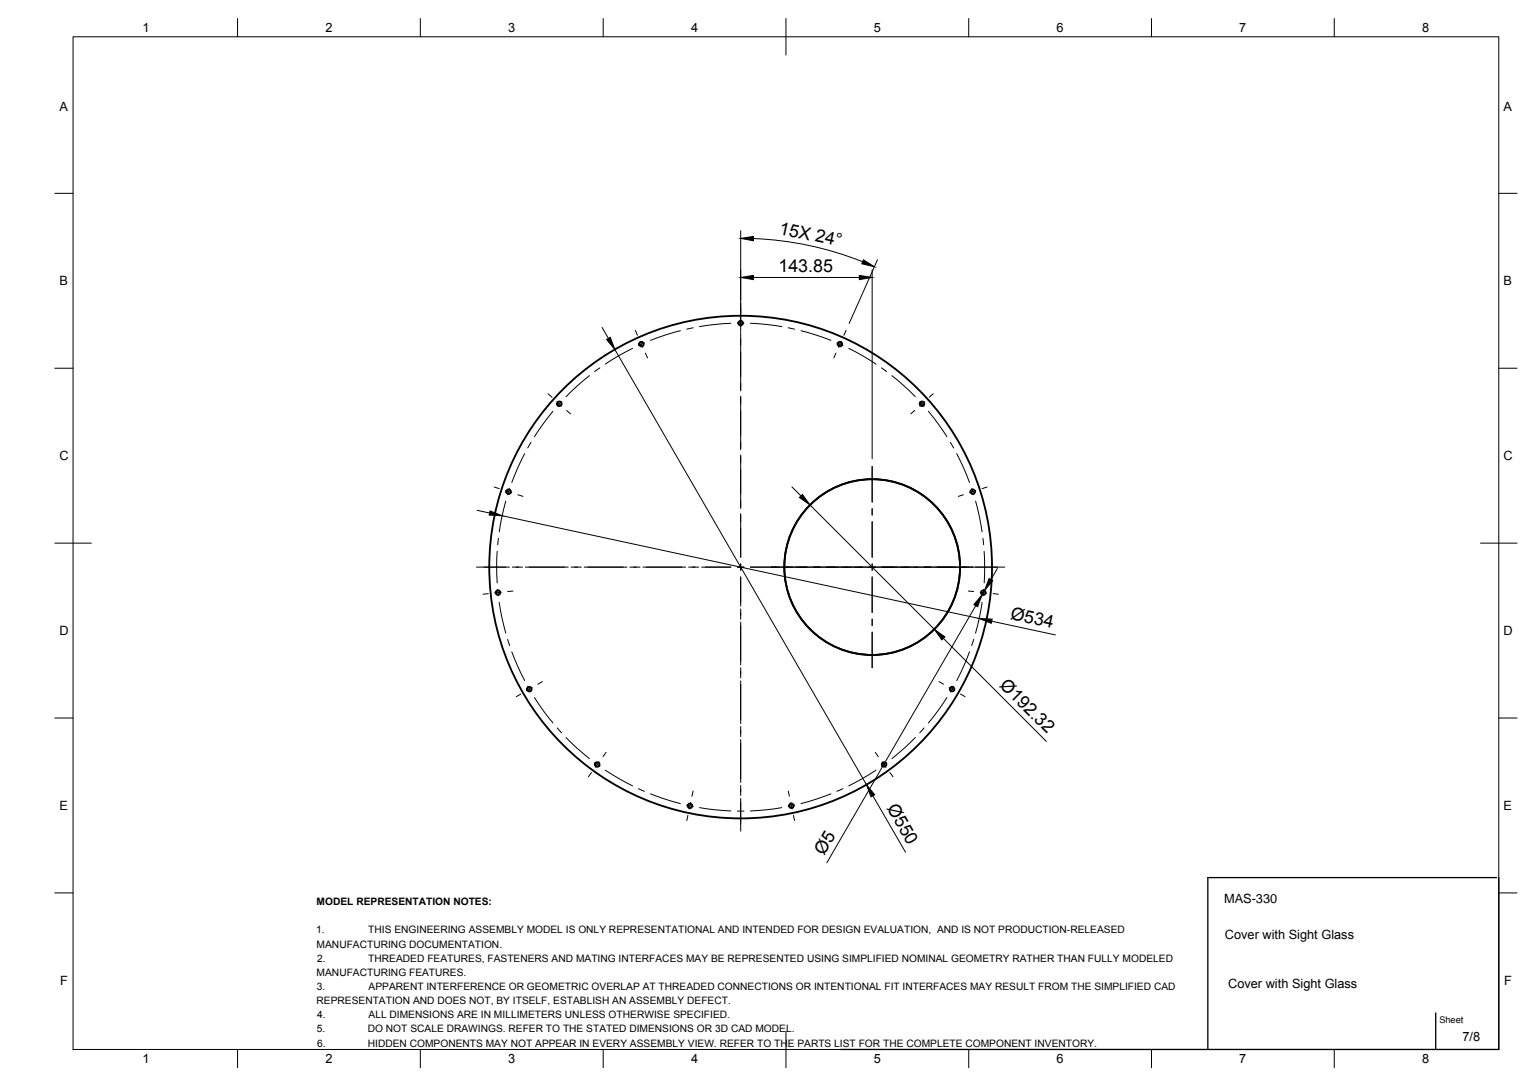
ISO-10303-21;
HEADER;
/* Generated by software containing ST-Developer
 * from STEP Tools, Inc. (www.steptools.com) 
 */

FILE_DESCRIPTION(
/* description */ ('STEP AP214'),
/* implementation_level */ '2;1');

FILE_NAME(
/* name */ 'Cover with Sight Glass.step',
/* time_stamp */ '2026-10-12T14:05:15-07:00',
/* author */ (''),
/* organization */ (''),
/* preprocessor_version */ 'ST-DEVELOPER v20.2',
/* originating_system */ 'Autodesk Translation Framework v15.15.0.0',
/* authorisation */ '');

FILE_SCHEMA (('AUTOMOTIVE_DESIGN { 1 0 10303 214 3 1 1 }'));
ENDSEC;

DATA;
#10=MECHANICAL_DESIGN_GEOMETRIC_PRESENTATION_REPRESENTATION('',(#286,#287),#39959);
#272=SHAPE_REPRESENTATION_RELATIONSHIP('SRR','None',#40006,#279);
#279=ADVANCED_BREP_SHAPE_REPRESENTATION('',(#294,#295),#39956);
#286=STYLED_ITEM('',(#40046),#294);
#287=STYLED_ITEM('',(#40046),#295);
#294=MANIFOLD_SOLID_BREP('Body1',#18263);
#295=MANIFOLD_SOLID_BREP('Body2',#18264);
#419=PLANE('',#18845);
#420=PLANE('',#18846);
#421=PLANE('',#18850);
#422=PLANE('',#18851);
#964=FACE_BOUND('',#6153,.T.);
#965=FACE_BOUND('',#6154,.T.);
#966=FACE_BOUND('',#6155,.T.);
#967=FACE_BOUND('',#6156,.T.);
#968=FACE_BOUND('',#6157,.T.);
#969=FACE_BOUND('',#6158,.T.);
#970=FACE_BOUND('',#6159,.T.);
#971=FACE_BOUND('',#6160,.T.);
#972=FACE_BOUND('',#6161,.T.);
#973=FACE_BOUND('',#6162,.T.);
#974=FACE_BOUND('',#6163,.T.);
#975=FACE_BOUND('',#6164,.T.);
#976=FACE_BOUND('',#6165,.T.);
#977=FACE_BOUND('',#6166,.T.);
#978=FACE_BOUND('',#6167,.T.);
#979=FACE_BOUND('',#6168,.T.);
#980=FACE_BOUND('',#6170,.T.);
#981=FACE_BOUND('',#6171,.T.);
#982=FACE_BOUND('',#6172,.T.);
#983=FACE_BOUND('',#6173,.T.);
#984=FACE_BOUND('',#6174,.T.);
#985=FACE_BOUND('',#6175,.T.);
#986=FACE_BOUND('',#6176,.T.);
#987=FACE_BOUND('',#6177,.T.);
#988=FACE_BOUND('',#6178,.T.);
#989=FACE_BOUND('',#6179,.T.);
#990=FACE_BOUND('',#6180,.T.);
#991=FACE_BOUND('',#6181,.T.);
#992=FACE_BOUND('',#6182,.T.);
#993=FACE_BOUND('',#6183,.T.);
#994=FACE_BOUND('',#6184,.T.);
#995=FACE_BOUND('',#6185,.T.);
#1772=LINE('',#30494,#3345);
#1773=LINE('',#30500,#3346);
#1774=LINE('',#30506,#3347);
#1775=LINE('',#30512,#3348);
#1776=LINE('',#30518,#3349);
#1777=LINE('',#30524,#3350);
#1778=LINE('',#30530,#3351);
#1779=LINE('',#30536,#3352);
#1780=LINE('',#30542,#3353);
#1781=LINE('',#30548,#3354);
#1782=LINE('',#30554,#3355);
#1783=LINE('',#30560,#3356);
#1784=LINE('',#30566,#3357);
#1785=LINE('',#30572,#3358);
#1786=LINE('',#30578,#3359);
#1787=LINE('',#30584,#3360);
#1788=LINE('',#30590,#3361);
#1789=LINE('',#30598,#3362);
#3345=VECTOR('',#21268,96.161193339026);
#3346=VECTOR('',#21275,2.5);
#3347=VECTOR('',#21282,2.5);
#3348=VECTOR('',#21289,2.5);
#3349=VECTOR('',#21296,2.5);
#3350=VECTOR('',#21303,2.5);
#3351=VECTOR('',#21310,2.5);
#3352=VECTOR('',#21317,2.5);
#3353=VECTOR('',#21324,2.5);
#3354=VECTOR('',#21331,2.50000000000001);
#3355=VECTOR('',#21338,2.5);
#3356=VECTOR('',#21345,2.5);
#3357=VECTOR('',#21352,2.5);
#3358=VECTOR('',#21359,2.5);
#3359=VECTOR('',#21366,2.5);
#3360=VECTOR('',#21373,2.5);
#3361=VECTOR('',#21380,275.);
#3362=VECTOR('',#21391,96.161193339026);
#4656=CYLINDRICAL_SURFACE('',#18794,96.161193339026);
#4657=CYLINDRICAL_SURFACE('',#18797,2.5);
#4658=CYLINDRICAL_SURFACE('',#18800,2.5);
#4659=CYLINDRICAL_SURFACE('',#18803,2.5);
#4660=CYLINDRICAL_SURFACE('',#18806,2.5);
#4661=CYLINDRICAL_SURFACE('',#18809,2.5);
#4662=CYLINDRICAL_SURFACE('',#18812,2.5);
#4663=CYLINDRICAL_SURFACE('',#18815,2.5);
#4664=CYLINDRICAL_SURFACE('',#18818,2.5);
#4665=CYLINDRICAL_SURFACE('',#18821,2.50000000000001);
#4666=CYLINDRICAL_SURFACE('',#18824,2.5);
#4667=CYLINDRICAL_SURFACE('',#18827,2.5);
#4668=CYLINDRICAL_SURFACE('',#18830,2.5);
#4669=CYLINDRICAL_SURFACE('',#18833,2.5);
#4670=CYLINDRICAL_SURFACE('',#18836,2.5);
#4671=CYLINDRICAL_SURFACE('',#18839,2.5);
#4672=CYLINDRICAL_SURFACE('',#18842,275.);
#4673=CYLINDRICAL_SURFACE('',#18847,96.161193339026);
#5054=FACE_OUTER_BOUND('',#6135,.T.);
#5055=FACE_OUTER_BOUND('',#6136,.T.);
#5056=FACE_OUTER_BOUND('',#6137,.T.);
#5057=FACE_OUTER_BOUND('',#6138,.T.);
#5058=FACE_OUTER_BOUND('',#6139,.T.);
#5059=FACE_OUTER_BOUND('',#6140,.T.);
#5060=FACE_OUTER_BOUND('',#6141,.T.);
#5061=FACE_OUTER_BOUND('',#6142,.T.);
#5062=FACE_OUTER_BOUND('',#6143,.T.);
#5063=FACE_OUTER_BOUND('',#6144,.T.);
#5064=FACE_OUTER_BOUND('',#6145,.T.);
#5065=FACE_OUTER_BOUND('',#6146,.T.);
#5066=FACE_OUTER_BOUND('',#6147,.T.);
#5067=FACE_OUTER_BOUND('',#6148,.T.);
#5068=FACE_OUTER_BOUND('',#6149,.T.);
#5069=FACE_OUTER_BOUND('',#6150,.T.);
#5070=FACE_OUTER_BOUND('',#6151,.T.);
#5071=FACE_OUTER_BOUND('',#6152,.T.);
#5072=FACE_OUTER_BOUND('',#6169,.T.);
#5073=FACE_OUTER_BOUND('',#6186,.T.);
#5074=FACE_OUTER_BOUND('',#6187,.T.);
#5075=FACE_OUTER_BOUND('',#6188,.T.);
#6135=EDGE_LOOP('',(#13262,#13263,#13264,#13265));
#6136=EDGE_LOOP('',(#13266,#13267,#13268,#13269));
#6137=EDGE_LOOP('',(#13270,#13271,#13272,#13273));
#6138=EDGE_LOOP('',(#13274,#13275,#13276,#13277));
#6139=EDGE_LOOP('',(#13278,#13279,#13280,#13281));
#6140=EDGE_LOOP('',(#13282,#13283,#13284,#13285));
#6141=EDGE_LOOP('',(#13286,#13287,#13288,#13289));
#6142=EDGE_LOOP('',(#13290,#13291,#13292,#13293));
#6143=EDGE_LOOP('',(#13294,#13295,#13296,#13297));
#6144=EDGE_LOOP('',(#13298,#13299,#13300,#13301));
#6145=EDGE_LOOP('',(#13302,#13303,#13304,#13305));
#6146=EDGE_LOOP('',(#13306,#13307,#13308,#13309));
#6147=EDGE_LOOP('',(#13310,#13311,#13312,#13313));
#6148=EDGE_LOOP('',(#13314,#13315,#13316,#13317));
#6149=EDGE_LOOP('',(#13318,#13319,#13320,#13321));
#6150=EDGE_LOOP('',(#13322,#13323,#13324,#13325));
#6151=EDGE_LOOP('',(#13326,#13327,#13328,#13329));
#6152=EDGE_LOOP('',(#13330));
#6153=EDGE_LOOP('',(#13331));
#6154=EDGE_LOOP('',(#13332));
#6155=EDGE_LOOP('',(#13333));
#6156=EDGE_LOOP('',(#13334));
#6157=EDGE_LOOP('',(#13335));
#6158=EDGE_LOOP('',(#13336));
#6159=EDGE_LOOP('',(#13337));
#6160=EDGE_LOOP('',(#13338));
#6161=EDGE_LOOP('',(#13339));
#6162=EDGE_LOOP('',(#13340));
#6163=EDGE_LOOP('',(#13341));
#6164=EDGE_LOOP('',(#13342));
#6165=EDGE_LOOP('',(#13343));
#6166=EDGE_LOOP('',(#13344));
#6167=EDGE_LOOP('',(#13345));
#6168=EDGE_LOOP('',(#13346));
#6169=EDGE_LOOP('',(#13347));
#6170=EDGE_LOOP('',(#13348));
#6171=EDGE_LOOP('',(#13349));
#6172=EDGE_LOOP('',(#13350));
#6173=EDGE_LOOP('',(#13351));
#6174=EDGE_LOOP('',(#13352));
#6175=EDGE_LOOP('',(#13353));
#6176=EDGE_LOOP('',(#13354));
#6177=EDGE_LOOP('',(#13355));
#6178=EDGE_LOOP('',(#13356));
#6179=EDGE_LOOP('',(#13357));
#6180=EDGE_LOOP('',(#13358));
#6181=EDGE_LOOP('',(#13359));
#6182=EDGE_LOOP('',(#13360));
#6183=EDGE_LOOP('',(#13361));
#6184=EDGE_LOOP('',(#13362));
#6185=EDGE_LOOP('',(#13363));
#6186=EDGE_LOOP('',(#13364,#13365,#13366,#13367));
#6187=EDGE_LOOP('',(#13368));
#6188=EDGE_LOOP('',(#13369));
#7199=CIRCLE('',#18795,96.161193339026);
#7200=CIRCLE('',#18796,96.161193339026);
#7201=CIRCLE('',#18798,2.5);
#7202=CIRCLE('',#18799,2.5);
#7203=CIRCLE('',#18801,2.5);
#7204=CIRCLE('',#18802,2.5);
#7205=CIRCLE('',#18804,2.5);
#7206=CIRCLE('',#18805,2.5);
#7207=CIRCLE('',#18807,2.5);
#7208=CIRCLE('',#18808,2.5);
#7209=CIRCLE('',#18810,2.5);
#7210=CIRCLE('',#18811,2.5);
#7211=CIRCLE('',#18813,2.5);
#7212=CIRCLE('',#18814,2.5);
#7213=CIRCLE('',#18816,2.5);
#7214=CIRCLE('',#18817,2.5);
#7215=CIRCLE('',#18819,2.5);
#7216=CIRCLE('',#18820,2.5);
#7217=CIRCLE('',#18822,2.50000000000001);
#7218=CIRCLE('',#18823,2.50000000000001);
#7219=CIRCLE('',#18825,2.5);
#7220=CIRCLE('',#18826,2.5);
#7221=CIRCLE('',#18828,2.5);
#7222=CIRCLE('',#18829,2.5);
#7223=CIRCLE('',#18831,2.5);
#7224=CIRCLE('',#18832,2.5);
#7225=CIRCLE('',#18834,2.5);
#7226=CIRCLE('',#18835,2.5);
#7227=CIRCLE('',#18837,2.5);
#7228=CIRCLE('',#18838,2.5);
#7229=CIRCLE('',#18840,2.5);
#7230=CIRCLE('',#18841,2.5);
#7231=CIRCLE('',#18843,275.);
#7232=CIRCLE('',#18844,275.);
#7233=CIRCLE('',#18848,96.161193339026);
#7234=CIRCLE('',#18849,96.161193339026);
#8086=VERTEX_POINT('',#30491);
#8087=VERTEX_POINT('',#30493);
#8088=VERTEX_POINT('',#30497);
#8089=VERTEX_POINT('',#30499);
#8090=VERTEX_POINT('',#30503);
#8091=VERTEX_POINT('',#30505);
#8092=VERTEX_POINT('',#30509);
#8093=VERTEX_POINT('',#30511);
#8094=VERTEX_POINT('',#30515);
#8095=VERTEX_POINT('',#30517);
#8096=VERTEX_POINT('',#30521);
#8097=VERTEX_POINT('',#30523);
#8098=VERTEX_POINT('',#30527);
#8099=VERTEX_POINT('',#30529);
#8100=VERTEX_POINT('',#30533);
#8101=VERTEX_POINT('',#30535);
#8102=VERTEX_POINT('',#30539);
#8103=VERTEX_POINT('',#30541);
#8104=VERTEX_POINT('',#30545);
#8105=VERTEX_POINT('',#30547);
#8106=VERTEX_POINT('',#30551);
#8107=VERTEX_POINT('',#30553);
#8108=VERTEX_POINT('',#30557);
#8109=VERTEX_POINT('',#30559);
#8110=VERTEX_POINT('',#30563);
#8111=VERTEX_POINT('',#30565);
#8112=VERTEX_POINT('',#30569);
#8113=VERTEX_POINT('',#30571);
#8114=VERTEX_POINT('',#30575);
#8115=VERTEX_POINT('',#30577);
#8116=VERTEX_POINT('',#30581);
#8117=VERTEX_POINT('',#30583);
#8118=VERTEX_POINT('',#30587);
#8119=VERTEX_POINT('',#30589);
#8120=VERTEX_POINT('',#30595);
#8121=VERTEX_POINT('',#30597);
#10011=EDGE_CURVE('',#8086,#8086,#7199,.T.);
#10012=EDGE_CURVE('',#8086,#8087,#1772,.T.);
#10013=EDGE_CURVE('',#8087,#8087,#7200,.T.);
#10014=EDGE_CURVE('',#8088,#8088,#7201,.T.);
#10015=EDGE_CURVE('',#8088,#8089,#1773,.T.);
#10016=EDGE_CURVE('',#8089,#8089,#7202,.T.);
#10017=EDGE_CURVE('',#8090,#8090,#7203,.T.);
#10018=EDGE_CURVE('',#8090,#8091,#1774,.T.);
#10019=EDGE_CURVE('',#8091,#8091,#7204,.T.);
#10020=EDGE_CURVE('',#8092,#8092,#7205,.T.);
#10021=EDGE_CURVE('',#8092,#8093,#1775,.T.);
#10022=EDGE_CURVE('',#8093,#8093,#7206,.T.);
#10023=EDGE_CURVE('',#8094,#8094,#7207,.T.);
#10024=EDGE_CURVE('',#8094,#8095,#1776,.T.);
#10025=EDGE_CURVE('',#8095,#8095,#7208,.T.);
#10026=EDGE_CURVE('',#8096,#8096,#7209,.T.);
#10027=EDGE_CURVE('',#8096,#8097,#1777,.T.);
#10028=EDGE_CURVE('',#8097,#8097,#7210,.T.);
#10029=EDGE_CURVE('',#8098,#8098,#7211,.T.);
#10030=EDGE_CURVE('',#8098,#8099,#1778,.T.);
#10031=EDGE_CURVE('',#8099,#8099,#7212,.T.);
#10032=EDGE_CURVE('',#8100,#8100,#7213,.T.);
#10033=EDGE_CURVE('',#8100,#8101,#1779,.T.);
#10034=EDGE_CURVE('',#8101,#8101,#7214,.T.);
#10035=EDGE_CURVE('',#8102,#8102,#7215,.T.);
#10036=EDGE_CURVE('',#8102,#8103,#1780,.T.);
#10037=EDGE_CURVE('',#8103,#8103,#7216,.T.);
#10038=EDGE_CURVE('',#8104,#8104,#7217,.T.);
#10039=EDGE_CURVE('',#8104,#8105,#1781,.T.);
#10040=EDGE_CURVE('',#8105,#8105,#7218,.T.);
#10041=EDGE_CURVE('',#8106,#8106,#7219,.T.);
#10042=EDGE_CURVE('',#8106,#8107,#1782,.T.);
#10043=EDGE_CURVE('',#8107,#8107,#7220,.T.);
#10044=EDGE_CURVE('',#8108,#8108,#7221,.T.);
#10045=EDGE_CURVE('',#8108,#8109,#1783,.T.);
#10046=EDGE_CURVE('',#8109,#8109,#7222,.T.);
#10047=EDGE_CURVE('',#8110,#8110,#7223,.T.);
#10048=EDGE_CURVE('',#8110,#8111,#1784,.T.);
#10049=EDGE_CURVE('',#8111,#8111,#7224,.T.);
#10050=EDGE_CURVE('',#8112,#8112,#7225,.T.);
#10051=EDGE_CURVE('',#8112,#8113,#1785,.T.);
#10052=EDGE_CURVE('',#8113,#8113,#7226,.T.);
#10053=EDGE_CURVE('',#8114,#8114,#7227,.T.);
#10054=EDGE_CURVE('',#8114,#8115,#1786,.T.);
#10055=EDGE_CURVE('',#8115,#8115,#7228,.T.);
#10056=EDGE_CURVE('',#8116,#8116,#7229,.T.);
#10057=EDGE_CURVE('',#8116,#8117,#1787,.T.);
#10058=EDGE_CURVE('',#8117,#8117,#7230,.T.);
#10059=EDGE_CURVE('',#8118,#8118,#7231,.T.);
#10060=EDGE_CURVE('',#8118,#8119,#1788,.T.);
#10061=EDGE_CURVE('',#8119,#8119,#7232,.T.);
#10062=EDGE_CURVE('',#8120,#8120,#7233,.T.);
#10063=EDGE_CURVE('',#8120,#8121,#1789,.T.);
#10064=EDGE_CURVE('',#8121,#8121,#7234,.T.);
#13262=ORIENTED_EDGE('',*,*,#10011,.F.);
#13263=ORIENTED_EDGE('',*,*,#10012,.T.);
#13264=ORIENTED_EDGE('',*,*,#10013,.T.);
#13265=ORIENTED_EDGE('',*,*,#10012,.F.);
#13266=ORIENTED_EDGE('',*,*,#10014,.T.);
#13267=ORIENTED_EDGE('',*,*,#10015,.T.);
#13268=ORIENTED_EDGE('',*,*,#10016,.F.);
#13269=ORIENTED_EDGE('',*,*,#10015,.F.);
#13270=ORIENTED_EDGE('',*,*,#10017,.T.);
#13271=ORIENTED_EDGE('',*,*,#10018,.T.);
#13272=ORIENTED_EDGE('',*,*,#10019,.F.);
#13273=ORIENTED_EDGE('',*,*,#10018,.F.);
#13274=ORIENTED_EDGE('',*,*,#10020,.T.);
#13275=ORIENTED_EDGE('',*,*,#10021,.T.);
#13276=ORIENTED_EDGE('',*,*,#10022,.F.);
#13277=ORIENTED_EDGE('',*,*,#10021,.F.);
#13278=ORIENTED_EDGE('',*,*,#10023,.T.);
#13279=ORIENTED_EDGE('',*,*,#10024,.T.);
#13280=ORIENTED_EDGE('',*,*,#10025,.F.);
#13281=ORIENTED_EDGE('',*,*,#10024,.F.);
#13282=ORIENTED_EDGE('',*,*,#10026,.T.);
#13283=ORIENTED_EDGE('',*,*,#10027,.T.);
#13284=ORIENTED_EDGE('',*,*,#10028,.F.);
#13285=ORIENTED_EDGE('',*,*,#10027,.F.);
#13286=ORIENTED_EDGE('',*,*,#10029,.T.);
#13287=ORIENTED_EDGE('',*,*,#10030,.T.);
#13288=ORIENTED_EDGE('',*,*,#10031,.F.);
#13289=ORIENTED_EDGE('',*,*,#10030,.F.);
#13290=ORIENTED_EDGE('',*,*,#10032,.T.);
#13291=ORIENTED_EDGE('',*,*,#10033,.T.);
#13292=ORIENTED_EDGE('',*,*,#10034,.F.);
#13293=ORIENTED_EDGE('',*,*,#10033,.F.);
#13294=ORIENTED_EDGE('',*,*,#10035,.T.);
#13295=ORIENTED_EDGE('',*,*,#10036,.T.);
#13296=ORIENTED_EDGE('',*,*,#10037,.F.);
#13297=ORIENTED_EDGE('',*,*,#10036,.F.);
#13298=ORIENTED_EDGE('',*,*,#10038,.T.);
#13299=ORIENTED_EDGE('',*,*,#10039,.T.);
#13300=ORIENTED_EDGE('',*,*,#10040,.F.);
#13301=ORIENTED_EDGE('',*,*,#10039,.F.);
#13302=ORIENTED_EDGE('',*,*,#10041,.T.);
#13303=ORIENTED_EDGE('',*,*,#10042,.T.);
#13304=ORIENTED_EDGE('',*,*,#10043,.F.);
#13305=ORIENTED_EDGE('',*,*,#10042,.F.);
#13306=ORIENTED_EDGE('',*,*,#10044,.T.);
#13307=ORIENTED_EDGE('',*,*,#10045,.T.);
#13308=ORIENTED_EDGE('',*,*,#10046,.F.);
#13309=ORIENTED_EDGE('',*,*,#10045,.F.);
#13310=ORIENTED_EDGE('',*,*,#10047,.T.);
#13311=ORIENTED_EDGE('',*,*,#10048,.T.);
#13312=ORIENTED_EDGE('',*,*,#10049,.F.);
#13313=ORIENTED_EDGE('',*,*,#10048,.F.);
#13314=ORIENTED_EDGE('',*,*,#10050,.T.);
#13315=ORIENTED_EDGE('',*,*,#10051,.T.);
#13316=ORIENTED_EDGE('',*,*,#10052,.F.);
#13317=ORIENTED_EDGE('',*,*,#10051,.F.);
#13318=ORIENTED_EDGE('',*,*,#10053,.T.);
#13319=ORIENTED_EDGE('',*,*,#10054,.T.);
#13320=ORIENTED_EDGE('',*,*,#10055,.F.);
#13321=ORIENTED_EDGE('',*,*,#10054,.F.);
#13322=ORIENTED_EDGE('',*,*,#10056,.T.);
#13323=ORIENTED_EDGE('',*,*,#10057,.T.);
#13324=ORIENTED_EDGE('',*,*,#10058,.F.);
#13325=ORIENTED_EDGE('',*,*,#10057,.F.);
#13326=ORIENTED_EDGE('',*,*,#10059,.T.);
#13327=ORIENTED_EDGE('',*,*,#10060,.T.);
#13328=ORIENTED_EDGE('',*,*,#10061,.F.);
#13329=ORIENTED_EDGE('',*,*,#10060,.F.);
#13330=ORIENTED_EDGE('',*,*,#10061,.T.);
#13331=ORIENTED_EDGE('',*,*,#10056,.F.);
#13332=ORIENTED_EDGE('',*,*,#10050,.F.);
#13333=ORIENTED_EDGE('',*,*,#10044,.F.);
#13334=ORIENTED_EDGE('',*,*,#10038,.F.);
#13335=ORIENTED_EDGE('',*,*,#10032,.F.);
#13336=ORIENTED_EDGE('',*,*,#10026,.F.);
#13337=ORIENTED_EDGE('',*,*,#10020,.F.);
#13338=ORIENTED_EDGE('',*,*,#10014,.F.);
#13339=ORIENTED_EDGE('',*,*,#10013,.F.);
#13340=ORIENTED_EDGE('',*,*,#10017,.F.);
#13341=ORIENTED_EDGE('',*,*,#10023,.F.);
#13342=ORIENTED_EDGE('',*,*,#10029,.F.);
#13343=ORIENTED_EDGE('',*,*,#10035,.F.);
#13344=ORIENTED_EDGE('',*,*,#10041,.F.);
#13345=ORIENTED_EDGE('',*,*,#10047,.F.);
#13346=ORIENTED_EDGE('',*,*,#10053,.F.);
#13347=ORIENTED_EDGE('',*,*,#10059,.F.);
#13348=ORIENTED_EDGE('',*,*,#10058,.T.);
#13349=ORIENTED_EDGE('',*,*,#10055,.T.);
#13350=ORIENTED_EDGE('',*,*,#10052,.T.);
#13351=ORIENTED_EDGE('',*,*,#10049,.T.);
#13352=ORIENTED_EDGE('',*,*,#10046,.T.);
#13353=ORIENTED_EDGE('',*,*,#10043,.T.);
#13354=ORIENTED_EDGE('',*,*,#10040,.T.);
#13355=ORIENTED_EDGE('',*,*,#10037,.T.);
#13356=ORIENTED_EDGE('',*,*,#10034,.T.);
#13357=ORIENTED_EDGE('',*,*,#10031,.T.);
#13358=ORIENTED_EDGE('',*,*,#10028,.T.);
#13359=ORIENTED_EDGE('',*,*,#10025,.T.);
#13360=ORIENTED_EDGE('',*,*,#10022,.T.);
#13361=ORIENTED_EDGE('',*,*,#10019,.T.);
#13362=ORIENTED_EDGE('',*,*,#10016,.T.);
#13363=ORIENTED_EDGE('',*,*,#10011,.T.);
#13364=ORIENTED_EDGE('',*,*,#10062,.F.);
#13365=ORIENTED_EDGE('',*,*,#10063,.T.);
#13366=ORIENTED_EDGE('',*,*,#10064,.T.);
#13367=ORIENTED_EDGE('',*,*,#10063,.F.);
#13368=ORIENTED_EDGE('',*,*,#10064,.F.);
#13369=ORIENTED_EDGE('',*,*,#10062,.T.);
#17498=ADVANCED_FACE('',(#5054),#4656,.F.);
#17499=ADVANCED_FACE('',(#5055),#4657,.F.);
#17500=ADVANCED_FACE('',(#5056),#4658,.F.);
#17501=ADVANCED_FACE('',(#5057),#4659,.F.);
#17502=ADVANCED_FACE('',(#5058),#4660,.F.);
#17503=ADVANCED_FACE('',(#5059),#4661,.F.);
#17504=ADVANCED_FACE('',(#5060),#4662,.F.);
#17505=ADVANCED_FACE('',(#5061),#4663,.F.);
#17506=ADVANCED_FACE('',(#5062),#4664,.F.);
#17507=ADVANCED_FACE('',(#5063),#4665,.F.);
#17508=ADVANCED_FACE('',(#5064),#4666,.F.);
#17509=ADVANCED_FACE('',(#5065),#4667,.F.);
#17510=ADVANCED_FACE('',(#5066),#4668,.F.);
#17511=ADVANCED_FACE('',(#5067),#4669,.F.);
#17512=ADVANCED_FACE('',(#5068),#4670,.F.);
#17513=ADVANCED_FACE('',(#5069),#4671,.F.);
#17514=ADVANCED_FACE('',(#5070),#4672,.T.);
#17515=ADVANCED_FACE('',(#5071,#964,#965,#966,#967,#968,#969,#970,#971,
#972,#973,#974,#975,#976,#977,#978,#979),#419,.T.);
#17516=ADVANCED_FACE('',(#5072,#980,#981,#982,#983,#984,#985,#986,#987,
#988,#989,#990,#991,#992,#993,#994,#995),#420,.F.);
#17517=ADVANCED_FACE('',(#5073),#4673,.T.);
#17518=ADVANCED_FACE('',(#5074),#421,.F.);
#17519=ADVANCED_FACE('',(#5075),#422,.T.);
#18263=CLOSED_SHELL('',(#17498,#17499,#17500,#17501,#17502,#17503,#17504,
#17505,#17506,#17507,#17508,#17509,#17510,#17511,#17512,#17513,#17514,#17515,
#17516));
#18264=CLOSED_SHELL('',(#17517,#17518,#17519));
#18793=AXIS2_PLACEMENT_3D('',#30489,#21262,#21263);
#18794=AXIS2_PLACEMENT_3D('',#30490,#21264,#21265);
#18795=AXIS2_PLACEMENT_3D('',#30492,#21266,#21267);
#18796=AXIS2_PLACEMENT_3D('',#30495,#21269,#21270);
#18797=AXIS2_PLACEMENT_3D('',#30496,#21271,#21272);
#18798=AXIS2_PLACEMENT_3D('',#30498,#21273,#21274);
#18799=AXIS2_PLACEMENT_3D('',#30501,#21276,#21277);
#18800=AXIS2_PLACEMENT_3D('',#30502,#21278,#21279);
#18801=AXIS2_PLACEMENT_3D('',#30504,#21280,#21281);
#18802=AXIS2_PLACEMENT_3D('',#30507,#21283,#21284);
#18803=AXIS2_PLACEMENT_3D('',#30508,#21285,#21286);
#18804=AXIS2_PLACEMENT_3D('',#30510,#21287,#21288);
#18805=AXIS2_PLACEMENT_3D('',#30513,#21290,#21291);
#18806=AXIS2_PLACEMENT_3D('',#30514,#21292,#21293);
#18807=AXIS2_PLACEMENT_3D('',#30516,#21294,#21295);
#18808=AXIS2_PLACEMENT_3D('',#30519,#21297,#21298);
#18809=AXIS2_PLACEMENT_3D('',#30520,#21299,#21300);
#18810=AXIS2_PLACEMENT_3D('',#30522,#21301,#21302);
#18811=AXIS2_PLACEMENT_3D('',#30525,#21304,#21305);
#18812=AXIS2_PLACEMENT_3D('',#30526,#21306,#21307);
#18813=AXIS2_PLACEMENT_3D('',#30528,#21308,#21309);
#18814=AXIS2_PLACEMENT_3D('',#30531,#21311,#21312);
#18815=AXIS2_PLACEMENT_3D('',#30532,#21313,#21314);
#18816=AXIS2_PLACEMENT_3D('',#30534,#21315,#21316);
#18817=AXIS2_PLACEMENT_3D('',#30537,#21318,#21319);
#18818=AXIS2_PLACEMENT_3D('',#30538,#21320,#21321);
#18819=AXIS2_PLACEMENT_3D('',#30540,#21322,#21323);
#18820=AXIS2_PLACEMENT_3D('',#30543,#21325,#21326);
#18821=AXIS2_PLACEMENT_3D('',#30544,#21327,#21328);
#18822=AXIS2_PLACEMENT_3D('',#30546,#21329,#21330);
#18823=AXIS2_PLACEMENT_3D('',#30549,#21332,#21333);
#18824=AXIS2_PLACEMENT_3D('',#30550,#21334,#21335);
#18825=AXIS2_PLACEMENT_3D('',#30552,#21336,#21337);
#18826=AXIS2_PLACEMENT_3D('',#30555,#21339,#21340);
#18827=AXIS2_PLACEMENT_3D('',#30556,#21341,#21342);
#18828=AXIS2_PLACEMENT_3D('',#30558,#21343,#21344);
#18829=AXIS2_PLACEMENT_3D('',#30561,#21346,#21347);
#18830=AXIS2_PLACEMENT_3D('',#30562,#21348,#21349);
#18831=AXIS2_PLACEMENT_3D('',#30564,#21350,#21351);
#18832=AXIS2_PLACEMENT_3D('',#30567,#21353,#21354);
#18833=AXIS2_PLACEMENT_3D('',#30568,#21355,#21356);
#18834=AXIS2_PLACEMENT_3D('',#30570,#21357,#21358);
#18835=AXIS2_PLACEMENT_3D('',#30573,#21360,#21361);
#18836=AXIS2_PLACEMENT_3D('',#30574,#21362,#21363);
#18837=AXIS2_PLACEMENT_3D('',#30576,#21364,#21365);
#18838=AXIS2_PLACEMENT_3D('',#30579,#21367,#21368);
#18839=AXIS2_PLACEMENT_3D('',#30580,#21369,#21370);
#18840=AXIS2_PLACEMENT_3D('',#30582,#21371,#21372);
#18841=AXIS2_PLACEMENT_3D('',#30585,#21374,#21375);
#18842=AXIS2_PLACEMENT_3D('',#30586,#21376,#21377);
#18843=AXIS2_PLACEMENT_3D('',#30588,#21378,#21379);
#18844=AXIS2_PLACEMENT_3D('',#30591,#21381,#21382);
#18845=AXIS2_PLACEMENT_3D('',#30592,#21383,#21384);
#18846=AXIS2_PLACEMENT_3D('',#30593,#21385,#21386);
#18847=AXIS2_PLACEMENT_3D('',#30594,#21387,#21388);
#18848=AXIS2_PLACEMENT_3D('',#30596,#21389,#21390);
#18849=AXIS2_PLACEMENT_3D('',#30599,#21392,#21393);
#18850=AXIS2_PLACEMENT_3D('',#30600,#21394,#21395);
#18851=AXIS2_PLACEMENT_3D('',#30601,#21396,#21397);
#21262=DIRECTION('axis',(0.,0.,1.));
#21263=DIRECTION('refdir',(1.,0.,0.));
#21264=DIRECTION('center_axis',(0.,0.,1.));
#21265=DIRECTION('ref_axis',(1.,0.,0.));
#21266=DIRECTION('center_axis',(0.,0.,1.));
#21267=DIRECTION('ref_axis',(1.,0.,0.));
#21268=DIRECTION('',(0.,0.,1.));
#21269=DIRECTION('center_axis',(0.,0.,1.));
#21270=DIRECTION('ref_axis',(1.,0.,0.));
#21271=DIRECTION('center_axis',(0.,0.,-1.));
#21272=DIRECTION('ref_axis',(-1.,0.,0.));
#21273=DIRECTION('center_axis',(0.,0.,1.));
#21274=DIRECTION('ref_axis',(1.,0.,0.));
#21275=DIRECTION('',(0.,0.,-1.));
#21276=DIRECTION('center_axis',(0.,0.,1.));
#21277=DIRECTION('ref_axis',(1.,0.,0.));
#21278=DIRECTION('center_axis',(0.,0.,-1.));
#21279=DIRECTION('ref_axis',(-1.,0.,0.));
#21280=DIRECTION('center_axis',(0.,0.,1.));
#21281=DIRECTION('ref_axis',(1.,0.,0.));
#21282=DIRECTION('',(0.,0.,-1.));
#21283=DIRECTION('center_axis',(0.,0.,1.));
#21284=DIRECTION('ref_axis',(1.,0.,0.));
#21285=DIRECTION('center_axis',(0.,0.,-1.));
#21286=DIRECTION('ref_axis',(-1.,0.,0.));
#21287=DIRECTION('center_axis',(0.,0.,1.));
#21288=DIRECTION('ref_axis',(1.,0.,0.));
#21289=DIRECTION('',(0.,0.,-1.));
#21290=DIRECTION('center_axis',(0.,0.,1.));
#21291=DIRECTION('ref_axis',(1.,0.,0.));
#21292=DIRECTION('center_axis',(0.,0.,-1.));
#21293=DIRECTION('ref_axis',(-1.,0.,0.));
#21294=DIRECTION('center_axis',(0.,0.,1.));
#21295=DIRECTION('ref_axis',(1.,0.,0.));
#21296=DIRECTION('',(0.,0.,-1.));
#21297=DIRECTION('center_axis',(0.,0.,1.));
#21298=DIRECTION('ref_axis',(1.,0.,0.));
#21299=DIRECTION('center_axis',(0.,0.,-1.));
#21300=DIRECTION('ref_axis',(-1.,0.,0.));
#21301=DIRECTION('center_axis',(0.,0.,1.));
#21302=DIRECTION('ref_axis',(1.,0.,0.));
#21303=DIRECTION('',(0.,0.,-1.));
#21304=DIRECTION('center_axis',(0.,0.,1.));
#21305=DIRECTION('ref_axis',(1.,0.,0.));
#21306=DIRECTION('center_axis',(0.,0.,-1.));
#21307=DIRECTION('ref_axis',(-1.,0.,0.));
#21308=DIRECTION('center_axis',(0.,0.,1.));
#21309=DIRECTION('ref_axis',(1.,0.,0.));
#21310=DIRECTION('',(0.,0.,-1.));
#21311=DIRECTION('center_axis',(0.,0.,1.));
#21312=DIRECTION('ref_axis',(1.,0.,0.));
#21313=DIRECTION('center_axis',(0.,0.,-1.));
#21314=DIRECTION('ref_axis',(-1.,0.,0.));
#21315=DIRECTION('center_axis',(0.,0.,1.));
#21316=DIRECTION('ref_axis',(1.,0.,0.));
#21317=DIRECTION('',(0.,0.,-1.));
#21318=DIRECTION('center_axis',(0.,0.,1.));
#21319=DIRECTION('ref_axis',(1.,0.,0.));
#21320=DIRECTION('center_axis',(0.,0.,-1.));
#21321=DIRECTION('ref_axis',(-1.,0.,0.));
#21322=DIRECTION('center_axis',(0.,0.,1.));
#21323=DIRECTION('ref_axis',(1.,0.,0.));
#21324=DIRECTION('',(0.,0.,-1.));
#21325=DIRECTION('center_axis',(0.,0.,1.));
#21326=DIRECTION('ref_axis',(1.,0.,0.));
#21327=DIRECTION('center_axis',(0.,0.,-1.));
#21328=DIRECTION('ref_axis',(-1.,0.,0.));
#21329=DIRECTION('center_axis',(0.,0.,1.));
#21330=DIRECTION('ref_axis',(1.,0.,0.));
#21331=DIRECTION('',(0.,0.,-1.));
#21332=DIRECTION('center_axis',(0.,0.,1.));
#21333=DIRECTION('ref_axis',(1.,0.,0.));
#21334=DIRECTION('center_axis',(0.,0.,-1.));
#21335=DIRECTION('ref_axis',(-1.,0.,0.));
#21336=DIRECTION('center_axis',(0.,0.,1.));
#21337=DIRECTION('ref_axis',(1.,0.,0.));
#21338=DIRECTION('',(0.,0.,-1.));
#21339=DIRECTION('center_axis',(0.,0.,1.));
#21340=DIRECTION('ref_axis',(1.,0.,0.));
#21341=DIRECTION('center_axis',(0.,0.,-1.));
#21342=DIRECTION('ref_axis',(-1.,0.,0.));
#21343=DIRECTION('center_axis',(0.,0.,1.));
#21344=DIRECTION('ref_axis',(1.,0.,0.));
#21345=DIRECTION('',(0.,0.,-1.));
#21346=DIRECTION('center_axis',(0.,0.,1.));
#21347=DIRECTION('ref_axis',(1.,0.,0.));
#21348=DIRECTION('center_axis',(0.,0.,-1.));
#21349=DIRECTION('ref_axis',(-1.,0.,0.));
#21350=DIRECTION('center_axis',(0.,0.,1.));
#21351=DIRECTION('ref_axis',(1.,0.,0.));
#21352=DIRECTION('',(0.,0.,-1.));
#21353=DIRECTION('center_axis',(0.,0.,1.));
#21354=DIRECTION('ref_axis',(1.,0.,0.));
#21355=DIRECTION('center_axis',(0.,0.,-1.));
#21356=DIRECTION('ref_axis',(-1.,0.,0.));
#21357=DIRECTION('center_axis',(0.,0.,1.));
#21358=DIRECTION('ref_axis',(1.,0.,0.));
#21359=DIRECTION('',(0.,0.,-1.));
#21360=DIRECTION('center_axis',(0.,0.,1.));
#21361=DIRECTION('ref_axis',(1.,0.,0.));
#21362=DIRECTION('center_axis',(0.,0.,-1.));
#21363=DIRECTION('ref_axis',(-1.,0.,0.));
#21364=DIRECTION('center_axis',(0.,0.,1.));
#21365=DIRECTION('ref_axis',(1.,0.,0.));
#21366=DIRECTION('',(0.,0.,-1.));
#21367=DIRECTION('center_axis',(0.,0.,1.));
#21368=DIRECTION('ref_axis',(1.,0.,0.));
#21369=DIRECTION('center_axis',(0.,0.,-1.));
#21370=DIRECTION('ref_axis',(-1.,0.,0.));
#21371=DIRECTION('center_axis',(0.,0.,1.));
#21372=DIRECTION('ref_axis',(1.,0.,0.));
#21373=DIRECTION('',(0.,0.,-1.));
#21374=DIRECTION('center_axis',(0.,0.,1.));
#21375=DIRECTION('ref_axis',(1.,0.,0.));
#21376=DIRECTION('center_axis',(0.,0.,-1.));
#21377=DIRECTION('ref_axis',(-1.,0.,0.));
#21378=DIRECTION('center_axis',(0.,0.,1.));
#21379=DIRECTION('ref_axis',(1.,0.,0.));
#21380=DIRECTION('',(0.,0.,1.));
#21381=DIRECTION('center_axis',(0.,0.,1.));
#21382=DIRECTION('ref_axis',(1.,0.,0.));
#21383=DIRECTION('center_axis',(0.,0.,1.));
#21384=DIRECTION('ref_axis',(1.,0.,0.));
#21385=DIRECTION('center_axis',(0.,0.,1.));
#21386=DIRECTION('ref_axis',(1.,0.,0.));
#21387=DIRECTION('center_axis',(0.,0.,1.));
#21388=DIRECTION('ref_axis',(1.,0.,0.));
#21389=DIRECTION('center_axis',(0.,0.,1.));
#21390=DIRECTION('ref_axis',(1.,0.,0.));
#21391=DIRECTION('',(0.,0.,-1.));
#21392=DIRECTION('center_axis',(0.,0.,1.));
#21393=DIRECTION('ref_axis',(1.,0.,0.));
#21394=DIRECTION('center_axis',(0.,0.,1.));
#21395=DIRECTION('ref_axis',(1.,0.,0.));
#21396=DIRECTION('center_axis',(0.,0.,1.));
#21397=DIRECTION('ref_axis',(1.,0.,0.));
#30489=CARTESIAN_POINT('',(0.,0.,0.));
#30490=CARTESIAN_POINT('Origin',(-143.851228669208,0.,55.));
#30491=CARTESIAN_POINT('',(-240.012422008234,-1.17763497624828E-14,55.));
#30492=CARTESIAN_POINT('Origin',(-143.851228669208,0.,55.));
#30493=CARTESIAN_POINT('',(-240.012422008234,-1.17763497624828E-14,60.));
#30494=CARTESIAN_POINT('',(-240.012422008234,-1.17763497624828E-14,55.));
#30495=CARTESIAN_POINT('Origin',(-143.851228669208,0.,60.));
#30496=CARTESIAN_POINT('Origin',(0.,267.,60.));
#30497=CARTESIAN_POINT('',(2.5,267.,60.));
#30498=CARTESIAN_POINT('Origin',(0.,267.,60.));
#30499=CARTESIAN_POINT('',(2.5,267.,55.));
#30500=CARTESIAN_POINT('',(2.5,267.,60.));
#30501=CARTESIAN_POINT('Origin',(0.,267.,55.));
#30502=CARTESIAN_POINT('Origin',(108.598683701239,243.916637190574,60.));
#30503=CARTESIAN_POINT('',(111.098683701239,243.916637190574,60.));
#30504=CARTESIAN_POINT('Origin',(108.598683701239,243.916637190574,60.));
#30505=CARTESIAN_POINT('',(111.098683701239,243.916637190574,55.));
#30506=CARTESIAN_POINT('',(111.098683701239,243.916637190574,60.));
#30507=CARTESIAN_POINT('Origin',(108.598683701239,243.916637190574,55.));
#30508=CARTESIAN_POINT('Origin',(198.419668402464,178.657871897815,60.));
#30509=CARTESIAN_POINT('',(200.919668402464,178.657871897815,60.));
#30510=CARTESIAN_POINT('Origin',(198.419668402464,178.657871897815,60.));
#30511=CARTESIAN_POINT('',(200.919668402464,178.657871897815,55.));
#30512=CARTESIAN_POINT('',(200.919668402464,178.657871897815,60.));
#30513=CARTESIAN_POINT('Origin',(198.419668402464,178.657871897815,55.));
#30514=CARTESIAN_POINT('Origin',(253.932089850806,82.507537498111,60.));
#30515=CARTESIAN_POINT('',(256.432089850806,82.507537498111,60.));
#30516=CARTESIAN_POINT('Origin',(253.932089850806,82.507537498111,60.));
#30517=CARTESIAN_POINT('',(256.432089850806,82.507537498111,55.));
#30518=CARTESIAN_POINT('',(256.432089850806,82.507537498111,60.));
#30519=CARTESIAN_POINT('Origin',(253.932089850806,82.507537498111,55.));
#30520=CARTESIAN_POINT('Origin',(265.537346063329,-27.9090996924634,60.));
#30521=CARTESIAN_POINT('',(268.037346063329,-27.9090996924634,60.));
#30522=CARTESIAN_POINT('Origin',(265.537346063329,-27.9090996924634,60.));
#30523=CARTESIAN_POINT('',(268.037346063329,-27.9090996924634,55.));
#30524=CARTESIAN_POINT('',(268.037346063329,-27.9090996924634,60.));
#30525=CARTESIAN_POINT('Origin',(265.537346063329,-27.9090996924634,55.));
#30526=CARTESIAN_POINT('Origin',(231.228782810445,-133.5,60.));
#30527=CARTESIAN_POINT('',(233.728782810445,-133.5,60.));
#30528=CARTESIAN_POINT('Origin',(231.228782810445,-133.5,60.));
#30529=CARTESIAN_POINT('',(233.728782810445,-133.5,55.));
#30530=CARTESIAN_POINT('',(233.728782810445,-133.5,60.));
#30531=CARTESIAN_POINT('Origin',(231.228782810445,-133.5,55.));
#30532=CARTESIAN_POINT('Origin',(156.93866236209,-216.007537498111,60.));
#30533=CARTESIAN_POINT('',(159.43866236209,-216.007537498111,60.));
#30534=CARTESIAN_POINT('Origin',(156.93866236209,-216.007537498111,60.));
#30535=CARTESIAN_POINT('',(159.43866236209,-216.007537498111,55.));
#30536=CARTESIAN_POINT('',(159.43866236209,-216.007537498111,60.));
#30537=CARTESIAN_POINT('Origin',(156.93866236209,-216.007537498111,55.));
#30538=CARTESIAN_POINT('Origin',(55.5124214483419,-261.165409395926,60.));
#30539=CARTESIAN_POINT('',(58.0124214483419,-261.165409395926,60.));
#30540=CARTESIAN_POINT('Origin',(55.5124214483419,-261.165409395926,60.));
#30541=CARTESIAN_POINT('',(58.0124214483419,-261.165409395926,55.));
#30542=CARTESIAN_POINT('',(58.0124214483419,-261.165409395926,60.));
#30543=CARTESIAN_POINT('Origin',(55.5124214483419,-261.165409395926,55.));
#30544=CARTESIAN_POINT('Origin',(-55.5124214483417,-261.165409395926,60.));
#30545=CARTESIAN_POINT('',(-53.0124214483417,-261.165409395926,60.));
#30546=CARTESIAN_POINT('Origin',(-55.5124214483417,-261.165409395926,60.));
#30547=CARTESIAN_POINT('',(-53.0124214483417,-261.165409395926,55.));
#30548=CARTESIAN_POINT('',(-53.0124214483417,-261.165409395926,60.));
#30549=CARTESIAN_POINT('Origin',(-55.5124214483417,-261.165409395926,55.));
#30550=CARTESIAN_POINT('Origin',(-156.93866236209,-216.007537498111,60.));
#30551=CARTESIAN_POINT('',(-154.43866236209,-216.007537498111,60.));
#30552=CARTESIAN_POINT('Origin',(-156.93866236209,-216.007537498111,60.));
#30553=CARTESIAN_POINT('',(-154.43866236209,-216.007537498111,55.));
#30554=CARTESIAN_POINT('',(-154.43866236209,-216.007537498111,60.));
#30555=CARTESIAN_POINT('Origin',(-156.93866236209,-216.007537498111,55.));
#30556=CARTESIAN_POINT('Origin',(-231.228782810445,-133.5,60.));
#30557=CARTESIAN_POINT('',(-228.728782810445,-133.5,60.));
#30558=CARTESIAN_POINT('Origin',(-231.228782810445,-133.5,60.));
#30559=CARTESIAN_POINT('',(-228.728782810445,-133.5,55.));
#30560=CARTESIAN_POINT('',(-228.728782810445,-133.5,60.));
#30561=CARTESIAN_POINT('Origin',(-231.228782810445,-133.5,55.));
#30562=CARTESIAN_POINT('Origin',(-265.537346063329,-27.9090996924637,60.));
#30563=CARTESIAN_POINT('',(-263.037346063329,-27.9090996924637,60.));
#30564=CARTESIAN_POINT('Origin',(-265.537346063329,-27.9090996924637,60.));
#30565=CARTESIAN_POINT('',(-263.037346063329,-27.9090996924637,55.));
#30566=CARTESIAN_POINT('',(-263.037346063329,-27.9090996924637,60.));
#30567=CARTESIAN_POINT('Origin',(-265.537346063329,-27.9090996924637,55.));
#30568=CARTESIAN_POINT('Origin',(-253.932089850806,82.5075374981109,60.));
#30569=CARTESIAN_POINT('',(-251.432089850806,82.5075374981109,60.));
#30570=CARTESIAN_POINT('Origin',(-253.932089850806,82.5075374981109,60.));
#30571=CARTESIAN_POINT('',(-251.432089850806,82.5075374981109,55.));
#30572=CARTESIAN_POINT('',(-251.432089850806,82.5075374981109,60.));
#30573=CARTESIAN_POINT('Origin',(-253.932089850806,82.5075374981109,55.));
#30574=CARTESIAN_POINT('Origin',(-198.419668402464,178.657871897815,60.));
#30575=CARTESIAN_POINT('',(-195.919668402464,178.657871897815,60.));
#30576=CARTESIAN_POINT('Origin',(-198.419668402464,178.657871897815,60.));
#30577=CARTESIAN_POINT('',(-195.919668402464,178.657871897815,55.));
#30578=CARTESIAN_POINT('',(-195.919668402464,178.657871897815,60.));
#30579=CARTESIAN_POINT('Origin',(-198.419668402464,178.657871897815,55.));
#30580=CARTESIAN_POINT('Origin',(-108.598683701239,243.916637190575,60.));
#30581=CARTESIAN_POINT('',(-106.098683701239,243.916637190575,60.));
#30582=CARTESIAN_POINT('Origin',(-108.598683701239,243.916637190575,60.));
#30583=CARTESIAN_POINT('',(-106.098683701239,243.916637190575,55.));
#30584=CARTESIAN_POINT('',(-106.098683701239,243.916637190575,60.));
#30585=CARTESIAN_POINT('Origin',(-108.598683701239,243.916637190575,55.));
#30586=CARTESIAN_POINT('Origin',(0.,0.,60.));
#30587=CARTESIAN_POINT('',(275.,-3.36777869765522E-14,55.));
#30588=CARTESIAN_POINT('Origin',(0.,0.,55.));
#30589=CARTESIAN_POINT('',(275.,-3.36777869765522E-14,60.));
#30590=CARTESIAN_POINT('',(275.,-3.36777869765522E-14,60.));
#30591=CARTESIAN_POINT('Origin',(0.,0.,60.));
#30592=CARTESIAN_POINT('Origin',(0.,0.,60.));
#30593=CARTESIAN_POINT('Origin',(0.,0.,55.));
#30594=CARTESIAN_POINT('Origin',(-143.851228669208,0.,55.));
#30595=CARTESIAN_POINT('',(-240.012422008234,-1.17763497624828E-14,60.));
#30596=CARTESIAN_POINT('Origin',(-143.851228669208,0.,60.));
#30597=CARTESIAN_POINT('',(-240.012422008234,-1.17763497624828E-14,55.));
#30598=CARTESIAN_POINT('',(-240.012422008234,-1.17763497624828E-14,55.));
#30599=CARTESIAN_POINT('Origin',(-143.851228669208,0.,55.));
#30600=CARTESIAN_POINT('Origin',(-143.851228669208,0.,55.));
#30601=CARTESIAN_POINT('Origin',(-143.851228669208,0.,60.));
#39947=UNCERTAINTY_MEASURE_WITH_UNIT(LENGTH_MEASURE(0.01),#39960,
'DISTANCE_ACCURACY_VALUE',
'Maximum model space distance between geometric entities at asserted c
onnectivities');
#39950=UNCERTAINTY_MEASURE_WITH_UNIT(LENGTH_MEASURE(0.01),#39960,
'DISTANCE_ACCURACY_VALUE',
'Maximum model space distance between geometric entities at asserted c
onnectivities');
#39956=(
GEOMETRIC_REPRESENTATION_CONTEXT(3)
GLOBAL_UNCERTAINTY_ASSIGNED_CONTEXT((#39947))
GLOBAL_UNIT_ASSIGNED_CONTEXT((#39960,#39962,#39963))
REPRESENTATION_CONTEXT('','3D')
);
#39959=(
GEOMETRIC_REPRESENTATION_CONTEXT(3)
GLOBAL_UNCERTAINTY_ASSIGNED_CONTEXT((#39950))
GLOBAL_UNIT_ASSIGNED_CONTEXT((#39960,#39962,#39963))
REPRESENTATION_CONTEXT('','3D')
);
#39960=(
LENGTH_UNIT()
NAMED_UNIT(*)
SI_UNIT(.MILLI.,.METRE.)
);
#39962=(
NAMED_UNIT(*)
PLANE_ANGLE_UNIT()
SI_UNIT($,.RADIAN.)
);
#39963=(
NAMED_UNIT(*)
SI_UNIT($,.STERADIAN.)
SOLID_ANGLE_UNIT()
);
#39969=SHAPE_DEFINITION_REPRESENTATION(#39977,#40006);
#39977=PRODUCT_DEFINITION_SHAPE('',$,#40015);
#40006=SHAPE_REPRESENTATION('',(#18793),#39956);
#40009=PRODUCT_DEFINITION_CONTEXT('part definition',#40035,'design');
#40015=PRODUCT_DEFINITION('Cover with Sight Glass',
'Cover with Sight Glass',#40023,#40009);
#40023=PRODUCT_DEFINITION_FORMATION('',$,#40042);
#40035=APPLICATION_CONTEXT(
'Core Data for Automotive Mechanical Design Process');
#40036=PRODUCT_CONTEXT('part definition',#40035,'mechanical');
#40042=PRODUCT('Cover with Sight Glass','Cover with Sight Glass',$,(#40036));
#40046=PRESENTATION_STYLE_ASSIGNMENT((#40048));
#40048=SURFACE_STYLE_USAGE(.BOTH.,#40050);
#40050=SURFACE_SIDE_STYLE('',(#40052));
#40052=SURFACE_STYLE_FILL_AREA(#40054);
#40054=FILL_AREA_STYLE('Opaque(202,209,238)',(#40056));
#40056=FILL_AREA_STYLE_COLOUR('Opaque(202,209,238)',#40058);
#40058=COLOUR_RGB('Opaque(202,209,238)', 0.66274510, 0.83137255, 0.94901961);
ENDSEC;
END-ISO-10303-21;
